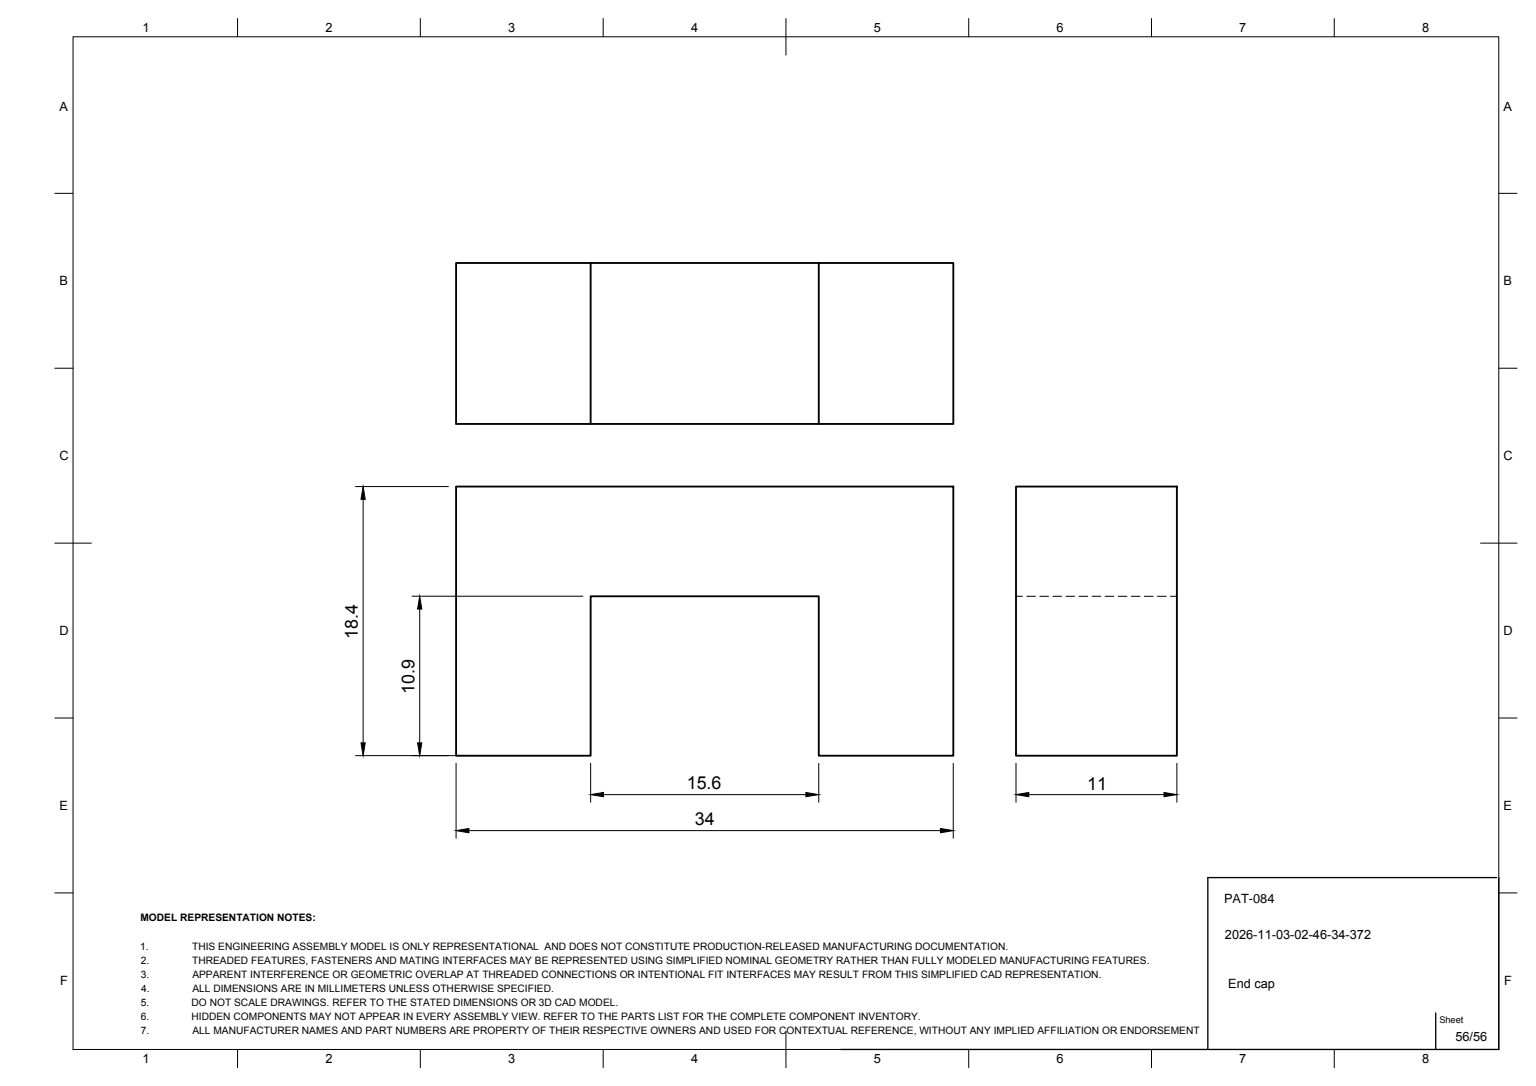
ISO-10303-21;
HEADER;
/* Generated by software containing ST-Developer
 * from STEP Tools, Inc. (www.steptools.com) 
 */

FILE_DESCRIPTION(
/* description */ ('Quick-return (Whitworth) mechanism'),
/* implementation_level */ '2;1');

FILE_NAME(
/* name */ 'End cap.step',
/* time_stamp */ '2026-10-28T03:25:57-07:00',
/* author */ (''),
/* organization */ (''),
/* preprocessor_version */ 'ST-DEVELOPER v20.2',
/* originating_system */ 'Autodesk Translation Framework v15.17.0.0',
/* authorisation */ '');

FILE_SCHEMA (('AUTOMOTIVE_DESIGN { 1 0 10303 214 3 1 1 }'));
ENDSEC;

DATA;
#10=MECHANICAL_DESIGN_GEOMETRIC_PRESENTATION_REPRESENTATION('',(#539),#14878);
#443=SHAPE_REPRESENTATION_RELATIONSHIP('SRR','None',#15118,#487);
#487=ADVANCED_BREP_SHAPE_REPRESENTATION('',(#590),#14875);
#539=STYLED_ITEM('',(#15420),#590);
#590=MANIFOLD_SOLID_BREP('Body1',#7894);
#1015=PLANE('',#9269);
#1016=PLANE('',#9270);
#1017=PLANE('',#9271);
#1018=PLANE('',#9272);
#1019=PLANE('',#9273);
#1020=PLANE('',#9274);
#1021=PLANE('',#9275);
#1022=PLANE('',#9276);
#1023=PLANE('',#9277);
#1024=PLANE('',#9278);
#1471=FACE_OUTER_BOUND('',#2126,.T.);
#1472=FACE_OUTER_BOUND('',#2127,.T.);
#1473=FACE_OUTER_BOUND('',#2128,.T.);
#1474=FACE_OUTER_BOUND('',#2129,.T.);
#1475=FACE_OUTER_BOUND('',#2130,.T.);
#1476=FACE_OUTER_BOUND('',#2131,.T.);
#1477=FACE_OUTER_BOUND('',#2132,.T.);
#1478=FACE_OUTER_BOUND('',#2133,.T.);
#1479=FACE_OUTER_BOUND('',#2134,.T.);
#1480=FACE_OUTER_BOUND('',#2135,.T.);
#2126=EDGE_LOOP('',(#7042,#7043,#7044,#7045));
#2127=EDGE_LOOP('',(#7046,#7047,#7048,#7049));
#2128=EDGE_LOOP('',(#7050,#7051,#7052,#7053));
#2129=EDGE_LOOP('',(#7054,#7055,#7056,#7057));
#2130=EDGE_LOOP('',(#7058,#7059,#7060,#7061));
#2131=EDGE_LOOP('',(#7062,#7063,#7064,#7065));
#2132=EDGE_LOOP('',(#7066,#7067,#7068,#7069));
#2133=EDGE_LOOP('',(#7070,#7071,#7072,#7073));
#2134=EDGE_LOOP('',(#7074,#7075,#7076,#7077,#7078,#7079,#7080,#7081));
#2135=EDGE_LOOP('',(#7082,#7083,#7084,#7085,#7086,#7087,#7088,#7089));
#2623=LINE('',#14522,#3146);
#2624=LINE('',#14524,#3147);
#2625=LINE('',#14526,#3148);
#2626=LINE('',#14527,#3149);
#2627=LINE('',#14530,#3150);
#2628=LINE('',#14532,#3151);
#2629=LINE('',#14533,#3152);
#2630=LINE('',#14536,#3153);
#2631=LINE('',#14538,#3154);
#2632=LINE('',#14539,#3155);
#2633=LINE('',#14542,#3156);
#2634=LINE('',#14544,#3157);
#2635=LINE('',#14545,#3158);
#2636=LINE('',#14548,#3159);
#2637=LINE('',#14550,#3160);
#2638=LINE('',#14551,#3161);
#2639=LINE('',#14554,#3162);
#2640=LINE('',#14556,#3163);
#2641=LINE('',#14557,#3164);
#2642=LINE('',#14560,#3165);
#2643=LINE('',#14562,#3166);
#2644=LINE('',#14563,#3167);
#2645=LINE('',#14565,#3168);
#2646=LINE('',#14566,#3169);
#3146=VECTOR('',#11622,1.);
#3147=VECTOR('',#11623,1.);
#3148=VECTOR('',#11624,1.);
#3149=VECTOR('',#11625,1.);
#3150=VECTOR('',#11628,1.);
#3151=VECTOR('',#11629,1.);
#3152=VECTOR('',#11630,1.);
#3153=VECTOR('',#11633,1.);
#3154=VECTOR('',#11634,1.);
#3155=VECTOR('',#11635,1.);
#3156=VECTOR('',#11638,1.);
#3157=VECTOR('',#11639,1.);
#3158=VECTOR('',#11640,1.);
#3159=VECTOR('',#11643,1.);
#3160=VECTOR('',#11644,1.);
#3161=VECTOR('',#11645,1.);
#3162=VECTOR('',#11648,1.);
#3163=VECTOR('',#11649,1.);
#3164=VECTOR('',#11650,1.);
#3165=VECTOR('',#11653,1.);
#3166=VECTOR('',#11654,1.);
#3167=VECTOR('',#11655,1.);
#3168=VECTOR('',#11658,1.);
#3169=VECTOR('',#11659,1.);
#4234=VERTEX_POINT('',#14520);
#4235=VERTEX_POINT('',#14521);
#4236=VERTEX_POINT('',#14523);
#4237=VERTEX_POINT('',#14525);
#4238=VERTEX_POINT('',#14529);
#4239=VERTEX_POINT('',#14531);
#4240=VERTEX_POINT('',#14535);
#4241=VERTEX_POINT('',#14537);
#4242=VERTEX_POINT('',#14541);
#4243=VERTEX_POINT('',#14543);
#4244=VERTEX_POINT('',#14547);
#4245=VERTEX_POINT('',#14549);
#4246=VERTEX_POINT('',#14553);
#4247=VERTEX_POINT('',#14555);
#4248=VERTEX_POINT('',#14559);
#4249=VERTEX_POINT('',#14561);
#5178=EDGE_CURVE('',#4234,#4235,#2623,.T.);
#5179=EDGE_CURVE('',#4234,#4236,#2624,.T.);
#5180=EDGE_CURVE('',#4237,#4236,#2625,.T.);
#5181=EDGE_CURVE('',#4235,#4237,#2626,.T.);
#5182=EDGE_CURVE('',#4235,#4238,#2627,.T.);
#5183=EDGE_CURVE('',#4239,#4237,#2628,.T.);
#5184=EDGE_CURVE('',#4238,#4239,#2629,.T.);
#5185=EDGE_CURVE('',#4238,#4240,#2630,.T.);
#5186=EDGE_CURVE('',#4241,#4239,#2631,.T.);
#5187=EDGE_CURVE('',#4240,#4241,#2632,.T.);
#5188=EDGE_CURVE('',#4240,#4242,#2633,.T.);
#5189=EDGE_CURVE('',#4243,#4241,#2634,.T.);
#5190=EDGE_CURVE('',#4242,#4243,#2635,.T.);
#5191=EDGE_CURVE('',#4242,#4244,#2636,.T.);
#5192=EDGE_CURVE('',#4245,#4243,#2637,.T.);
#5193=EDGE_CURVE('',#4244,#4245,#2638,.T.);
#5194=EDGE_CURVE('',#4244,#4246,#2639,.T.);
#5195=EDGE_CURVE('',#4247,#4245,#2640,.T.);
#5196=EDGE_CURVE('',#4246,#4247,#2641,.T.);
#5197=EDGE_CURVE('',#4246,#4248,#2642,.T.);
#5198=EDGE_CURVE('',#4249,#4247,#2643,.T.);
#5199=EDGE_CURVE('',#4248,#4249,#2644,.T.);
#5200=EDGE_CURVE('',#4248,#4234,#2645,.T.);
#5201=EDGE_CURVE('',#4236,#4249,#2646,.T.);
#7042=ORIENTED_EDGE('',*,*,#5178,.F.);
#7043=ORIENTED_EDGE('',*,*,#5179,.T.);
#7044=ORIENTED_EDGE('',*,*,#5180,.F.);
#7045=ORIENTED_EDGE('',*,*,#5181,.F.);
#7046=ORIENTED_EDGE('',*,*,#5182,.F.);
#7047=ORIENTED_EDGE('',*,*,#5181,.T.);
#7048=ORIENTED_EDGE('',*,*,#5183,.F.);
#7049=ORIENTED_EDGE('',*,*,#5184,.F.);
#7050=ORIENTED_EDGE('',*,*,#5185,.F.);
#7051=ORIENTED_EDGE('',*,*,#5184,.T.);
#7052=ORIENTED_EDGE('',*,*,#5186,.F.);
#7053=ORIENTED_EDGE('',*,*,#5187,.F.);
#7054=ORIENTED_EDGE('',*,*,#5188,.F.);
#7055=ORIENTED_EDGE('',*,*,#5187,.T.);
#7056=ORIENTED_EDGE('',*,*,#5189,.F.);
#7057=ORIENTED_EDGE('',*,*,#5190,.F.);
#7058=ORIENTED_EDGE('',*,*,#5191,.F.);
#7059=ORIENTED_EDGE('',*,*,#5190,.T.);
#7060=ORIENTED_EDGE('',*,*,#5192,.F.);
#7061=ORIENTED_EDGE('',*,*,#5193,.F.);
#7062=ORIENTED_EDGE('',*,*,#5194,.F.);
#7063=ORIENTED_EDGE('',*,*,#5193,.T.);
#7064=ORIENTED_EDGE('',*,*,#5195,.F.);
#7065=ORIENTED_EDGE('',*,*,#5196,.F.);
#7066=ORIENTED_EDGE('',*,*,#5197,.F.);
#7067=ORIENTED_EDGE('',*,*,#5196,.T.);
#7068=ORIENTED_EDGE('',*,*,#5198,.F.);
#7069=ORIENTED_EDGE('',*,*,#5199,.F.);
#7070=ORIENTED_EDGE('',*,*,#5200,.F.);
#7071=ORIENTED_EDGE('',*,*,#5199,.T.);
#7072=ORIENTED_EDGE('',*,*,#5201,.F.);
#7073=ORIENTED_EDGE('',*,*,#5179,.F.);
#7074=ORIENTED_EDGE('',*,*,#5200,.T.);
#7075=ORIENTED_EDGE('',*,*,#5178,.T.);
#7076=ORIENTED_EDGE('',*,*,#5182,.T.);
#7077=ORIENTED_EDGE('',*,*,#5185,.T.);
#7078=ORIENTED_EDGE('',*,*,#5188,.T.);
#7079=ORIENTED_EDGE('',*,*,#5191,.T.);
#7080=ORIENTED_EDGE('',*,*,#5194,.T.);
#7081=ORIENTED_EDGE('',*,*,#5197,.T.);
#7082=ORIENTED_EDGE('',*,*,#5201,.T.);
#7083=ORIENTED_EDGE('',*,*,#5198,.T.);
#7084=ORIENTED_EDGE('',*,*,#5195,.T.);
#7085=ORIENTED_EDGE('',*,*,#5192,.T.);
#7086=ORIENTED_EDGE('',*,*,#5189,.T.);
#7087=ORIENTED_EDGE('',*,*,#5186,.T.);
#7088=ORIENTED_EDGE('',*,*,#5183,.T.);
#7089=ORIENTED_EDGE('',*,*,#5180,.T.);
#7802=ADVANCED_FACE('',(#1471),#1015,.T.);
#7803=ADVANCED_FACE('',(#1472),#1016,.T.);
#7804=ADVANCED_FACE('',(#1473),#1017,.T.);
#7805=ADVANCED_FACE('',(#1474),#1018,.T.);
#7806=ADVANCED_FACE('',(#1475),#1019,.T.);
#7807=ADVANCED_FACE('',(#1476),#1020,.T.);
#7808=ADVANCED_FACE('',(#1477),#1021,.T.);
#7809=ADVANCED_FACE('',(#1478),#1022,.T.);
#7810=ADVANCED_FACE('',(#1479),#1023,.T.);
#7811=ADVANCED_FACE('',(#1480),#1024,.T.);
#7894=CLOSED_SHELL('',(#7802,#7803,#7804,#7805,#7806,#7807,#7808,#7809,
#7810,#7811));
#9268=AXIS2_PLACEMENT_3D('',#14518,#11618,#11619);
#9269=AXIS2_PLACEMENT_3D('',#14519,#11620,#11621);
#9270=AXIS2_PLACEMENT_3D('',#14528,#11626,#11627);
#9271=AXIS2_PLACEMENT_3D('',#14534,#11631,#11632);
#9272=AXIS2_PLACEMENT_3D('',#14540,#11636,#11637);
#9273=AXIS2_PLACEMENT_3D('',#14546,#11641,#11642);
#9274=AXIS2_PLACEMENT_3D('',#14552,#11646,#11647);
#9275=AXIS2_PLACEMENT_3D('',#14558,#11651,#11652);
#9276=AXIS2_PLACEMENT_3D('',#14564,#11656,#11657);
#9277=AXIS2_PLACEMENT_3D('',#14567,#11660,#11661);
#9278=AXIS2_PLACEMENT_3D('',#14568,#11662,#11663);
#11618=DIRECTION('axis',(0.,0.,1.));
#11619=DIRECTION('refdir',(1.,0.,0.));
#11620=DIRECTION('center_axis',(0.,0.,-1.));
#11621=DIRECTION('ref_axis',(0.,-1.,0.));
#11622=DIRECTION('',(0.,1.,0.));
#11623=DIRECTION('',(-1.,0.,0.));
#11624=DIRECTION('',(0.,-1.,0.));
#11625=DIRECTION('',(-1.,0.,0.));
#11626=DIRECTION('center_axis',(0.,1.,0.));
#11627=DIRECTION('ref_axis',(0.,0.,-1.));
#11628=DIRECTION('',(0.,0.,1.));
#11629=DIRECTION('',(0.,0.,-1.));
#11630=DIRECTION('',(-1.,0.,0.));
#11631=DIRECTION('center_axis',(0.,0.,-1.));
#11632=DIRECTION('ref_axis',(0.,-1.,0.));
#11633=DIRECTION('',(0.,1.,0.));
#11634=DIRECTION('',(0.,-1.,0.));
#11635=DIRECTION('',(-1.,0.,0.));
#11636=DIRECTION('center_axis',(0.,-1.,0.));
#11637=DIRECTION('ref_axis',(0.,0.,1.));
#11638=DIRECTION('',(0.,0.,-1.));
#11639=DIRECTION('',(0.,0.,1.));
#11640=DIRECTION('',(-1.,0.,0.));
#11641=DIRECTION('center_axis',(0.,0.,-1.));
#11642=DIRECTION('ref_axis',(0.,-1.,0.));
#11643=DIRECTION('',(0.,1.,0.));
#11644=DIRECTION('',(0.,-1.,0.));
#11645=DIRECTION('',(-1.,0.,0.));
#11646=DIRECTION('center_axis',(0.,1.,0.));
#11647=DIRECTION('ref_axis',(0.,0.,-1.));
#11648=DIRECTION('',(0.,0.,1.));
#11649=DIRECTION('',(0.,0.,-1.));
#11650=DIRECTION('',(-1.,0.,0.));
#11651=DIRECTION('center_axis',(0.,0.,1.));
#11652=DIRECTION('ref_axis',(0.,1.,0.));
#11653=DIRECTION('',(0.,-1.,0.));
#11654=DIRECTION('',(0.,1.,0.));
#11655=DIRECTION('',(-1.,0.,0.));
#11656=DIRECTION('center_axis',(0.,-1.,0.));
#11657=DIRECTION('ref_axis',(0.,0.,1.));
#11658=DIRECTION('',(0.,0.,-1.));
#11659=DIRECTION('',(0.,0.,1.));
#11660=DIRECTION('center_axis',(1.,0.,0.));
#11661=DIRECTION('ref_axis',(0.,0.,-1.));
#11662=DIRECTION('center_axis',(-1.,0.,0.));
#11663=DIRECTION('ref_axis',(0.,0.,1.));
#14518=CARTESIAN_POINT('',(0.,0.,0.));
#14519=CARTESIAN_POINT('Origin',(-1.97,-0.78,0.46));
#14520=CARTESIAN_POINT('',(-1.97,-1.7,0.46));
#14521=CARTESIAN_POINT('',(-1.97,-0.78,0.46));
#14522=CARTESIAN_POINT('',(-1.97,-1.7,0.46));
#14523=CARTESIAN_POINT('',(-3.07,-1.7,0.46));
#14524=CARTESIAN_POINT('',(-1.97,-1.7,0.46));
#14525=CARTESIAN_POINT('',(-3.07,-0.78,0.46));
#14526=CARTESIAN_POINT('',(-3.07,-1.7,0.46));
#14527=CARTESIAN_POINT('',(-1.97,-0.78,0.46));
#14528=CARTESIAN_POINT('Origin',(-1.97,-0.78,1.55));
#14529=CARTESIAN_POINT('',(-1.97,-0.78,1.55));
#14530=CARTESIAN_POINT('',(-1.97,-0.78,0.46));
#14531=CARTESIAN_POINT('',(-3.07,-0.78,1.55));
#14532=CARTESIAN_POINT('',(-3.07,-0.78,0.46));
#14533=CARTESIAN_POINT('',(-1.97,-0.78,1.55));
#14534=CARTESIAN_POINT('Origin',(-1.97,0.78,1.55));
#14535=CARTESIAN_POINT('',(-1.97,0.78,1.55));
#14536=CARTESIAN_POINT('',(-1.97,-0.78,1.55));
#14537=CARTESIAN_POINT('',(-3.07,0.78,1.55));
#14538=CARTESIAN_POINT('',(-3.07,-0.78,1.55));
#14539=CARTESIAN_POINT('',(-1.97,0.78,1.55));
#14540=CARTESIAN_POINT('Origin',(-1.97,0.78,0.46));
#14541=CARTESIAN_POINT('',(-1.97,0.78,0.46));
#14542=CARTESIAN_POINT('',(-1.97,0.78,1.55));
#14543=CARTESIAN_POINT('',(-3.07,0.78,0.46));
#14544=CARTESIAN_POINT('',(-3.07,0.78,1.55));
#14545=CARTESIAN_POINT('',(-1.97,0.78,0.46));
#14546=CARTESIAN_POINT('Origin',(-1.97,1.7,0.46));
#14547=CARTESIAN_POINT('',(-1.97,1.7,0.46));
#14548=CARTESIAN_POINT('',(-1.97,0.78,0.46));
#14549=CARTESIAN_POINT('',(-3.07,1.7,0.46));
#14550=CARTESIAN_POINT('',(-3.07,0.78,0.46));
#14551=CARTESIAN_POINT('',(-1.97,1.7,0.46));
#14552=CARTESIAN_POINT('Origin',(-1.97,1.7,2.3));
#14553=CARTESIAN_POINT('',(-1.97,1.7,2.3));
#14554=CARTESIAN_POINT('',(-1.97,1.7,0.46));
#14555=CARTESIAN_POINT('',(-3.07,1.7,2.3));
#14556=CARTESIAN_POINT('',(-3.07,1.7,0.46));
#14557=CARTESIAN_POINT('',(-1.97,1.7,2.3));
#14558=CARTESIAN_POINT('Origin',(-1.97,-1.7,2.3));
#14559=CARTESIAN_POINT('',(-1.97,-1.7,2.3));
#14560=CARTESIAN_POINT('',(-1.97,1.7,2.3));
#14561=CARTESIAN_POINT('',(-3.07,-1.7,2.3));
#14562=CARTESIAN_POINT('',(-3.07,1.7,2.3));
#14563=CARTESIAN_POINT('',(-1.97,-1.7,2.3));
#14564=CARTESIAN_POINT('Origin',(-1.97,-1.7,0.46));
#14565=CARTESIAN_POINT('',(-1.97,-1.7,2.3));
#14566=CARTESIAN_POINT('',(-3.07,-1.7,2.3));
#14567=CARTESIAN_POINT('Origin',(-1.97,0.,1.38));
#14568=CARTESIAN_POINT('Origin',(-3.07,0.,1.38));
#14821=UNCERTAINTY_MEASURE_WITH_UNIT(LENGTH_MEASURE(0.001),#14879,
'DISTANCE_ACCURACY_VALUE',
'Maximum model space distance between geometric entities at asserted c
onnectivities');
#14824=UNCERTAINTY_MEASURE_WITH_UNIT(LENGTH_MEASURE(0.001),#14879,
'DISTANCE_ACCURACY_VALUE',
'Maximum model space distance between geometric entities at asserted c
onnectivities');
#14875=(
GEOMETRIC_REPRESENTATION_CONTEXT(3)
GLOBAL_UNCERTAINTY_ASSIGNED_CONTEXT((#14821))
GLOBAL_UNIT_ASSIGNED_CONTEXT((#14879,#14881,#14882))
REPRESENTATION_CONTEXT('','3D')
);
#14878=(
GEOMETRIC_REPRESENTATION_CONTEXT(3)
GLOBAL_UNCERTAINTY_ASSIGNED_CONTEXT((#14824))
GLOBAL_UNIT_ASSIGNED_CONTEXT((#14879,#14881,#14882))
REPRESENTATION_CONTEXT('','3D')
);
#14879=(
LENGTH_UNIT()
NAMED_UNIT(*)
SI_UNIT(.CENTI.,.METRE.)
);
#14881=(
NAMED_UNIT(*)
PLANE_ANGLE_UNIT()
SI_UNIT($,.RADIAN.)
);
#14882=(
NAMED_UNIT(*)
SI_UNIT($,.STERADIAN.)
SOLID_ANGLE_UNIT()
);
#14933=SHAPE_DEFINITION_REPRESENTATION(#14995,#15118);
#14995=PRODUCT_DEFINITION_SHAPE('',$,#15172);
#15118=SHAPE_REPRESENTATION('',(#9268),#14875);
#15121=PRODUCT_DEFINITION_CONTEXT('part definition',#15282,'design');
#15172=PRODUCT_DEFINITION('End cap','End cap',#15225,#15121);
#15225=PRODUCT_DEFINITION_FORMATION('',$,#15334);
#15282=APPLICATION_CONTEXT(
'Core Data for Automotive Mechanical Design Process');
#15283=PRODUCT_CONTEXT('part definition',#15282,'mechanical');
#15334=PRODUCT('End cap','End cap','End cap',(#15283));
#15414=COLOUR_RGB('Off White',0.89,0.88,0.83);
#15415=FILL_AREA_STYLE_COLOUR('',#15414);
#15416=FILL_AREA_STYLE('',(#15415));
#15417=SURFACE_STYLE_FILL_AREA(#15416);
#15418=SURFACE_SIDE_STYLE('',(#15417));
#15419=SURFACE_STYLE_USAGE(.BOTH.,#15418);
#15420=PRESENTATION_STYLE_ASSIGNMENT((#15419));
ENDSEC;
END-ISO-10303-21;
